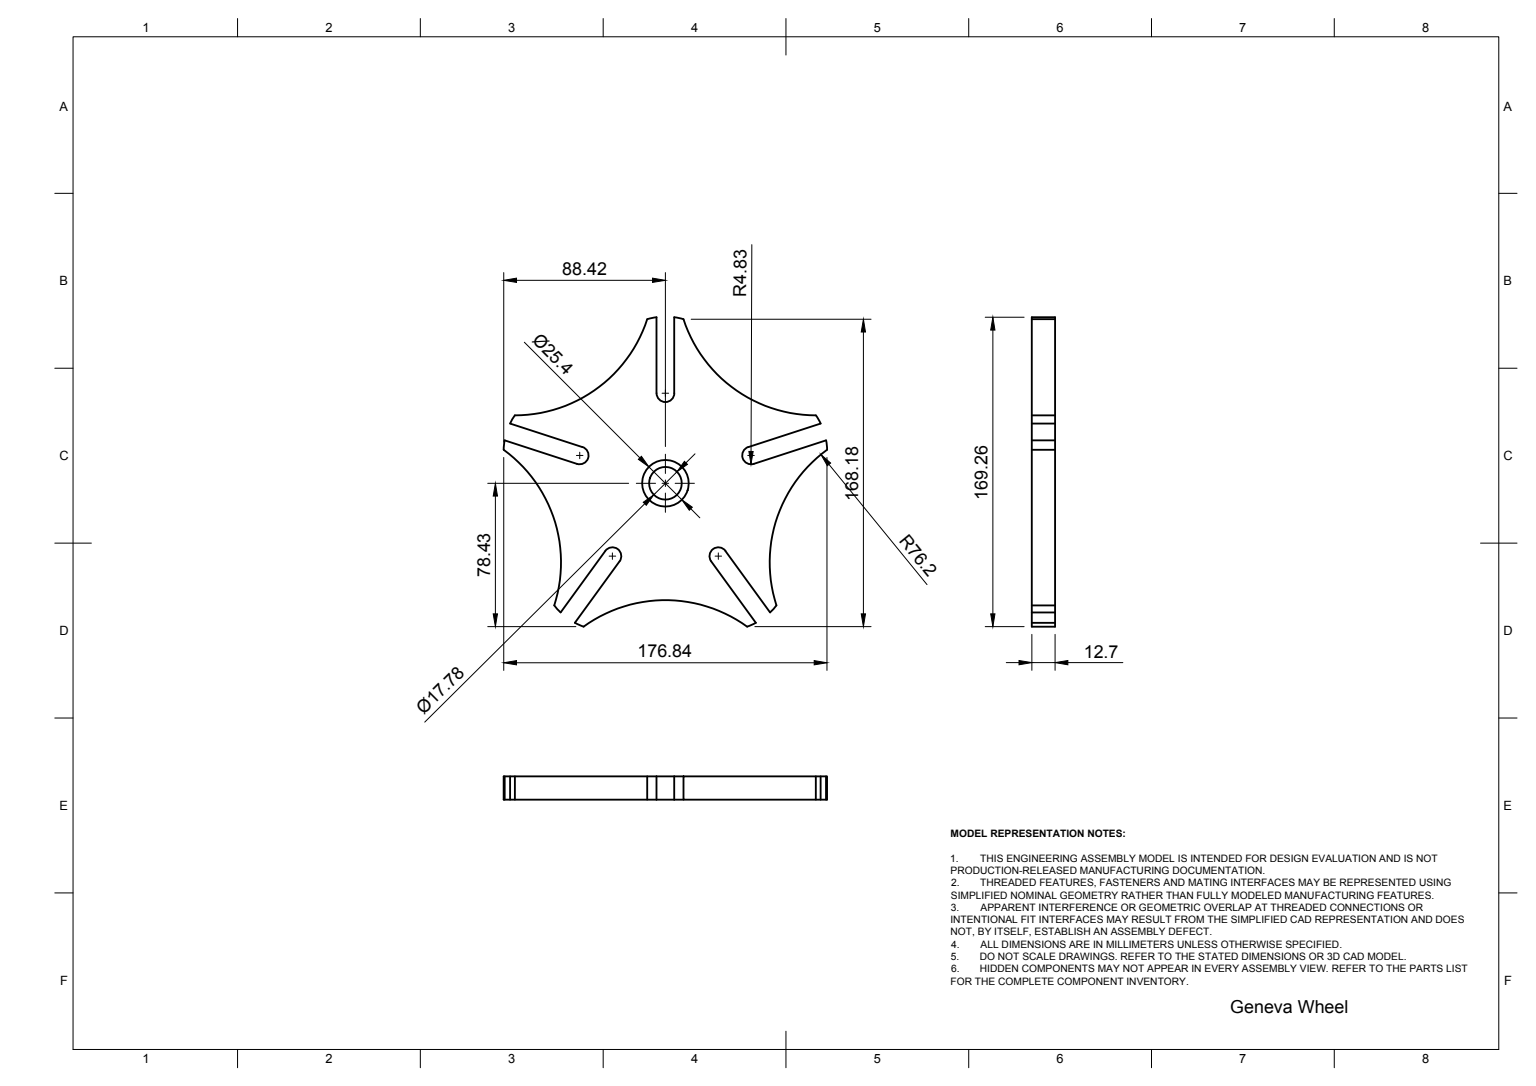
ISO-10303-21;
HEADER;
/* Generated by software containing ST-Developer
 * from STEP Tools, Inc. (www.steptools.com) 
 */

FILE_DESCRIPTION(
/* description */ ('STEP AP214'),
/* implementation_level */ '2;1');

FILE_NAME(
/* name */ 'Geneva Wheel.step',
/* time_stamp */ '2026-10-06T11:20:11-07:00',
/* author */ (''),
/* organization */ (''),
/* preprocessor_version */ 'ST-DEVELOPER v20.2',
/* originating_system */ 'Autodesk Translation Framework v15.15.0.0',
/* authorisation */ '');

FILE_SCHEMA (('AUTOMOTIVE_DESIGN { 1 0 10303 214 3 1 1 }'));
ENDSEC;

DATA;
#10=MECHANICAL_DESIGN_GEOMETRIC_PRESENTATION_REPRESENTATION('',(#51),#2840);
#39=SHAPE_REPRESENTATION_RELATIONSHIP('SRR','None',#2870,#45);
#45=ADVANCED_BREP_SHAPE_REPRESENTATION('',(#57),#2838);
#51=STYLED_ITEM('',(#2905),#57);
#57=MANIFOLD_SOLID_BREP('Body1',#1551);
#95=FACE_BOUND('',#299,.T.);
#96=FACE_BOUND('',#301,.T.);
#97=FACE_BOUND('',#330,.T.);
#111=PLANE('',#1765);
#112=PLANE('',#1783);
#113=PLANE('',#1802);
#114=PLANE('',#1806);
#115=PLANE('',#1808);
#116=PLANE('',#1812);
#117=PLANE('',#1813);
#118=PLANE('',#1816);
#119=PLANE('',#1817);
#120=PLANE('',#1821);
#121=PLANE('',#1823);
#122=PLANE('',#1827);
#123=PLANE('',#1828);
#178=FACE_OUTER_BOUND('',#293,.T.);
#179=FACE_OUTER_BOUND('',#294,.T.);
#180=FACE_OUTER_BOUND('',#295,.T.);
#181=FACE_OUTER_BOUND('',#296,.T.);
#182=FACE_OUTER_BOUND('',#297,.T.);
#183=FACE_OUTER_BOUND('',#298,.T.);
#184=FACE_OUTER_BOUND('',#300,.T.);
#185=FACE_OUTER_BOUND('',#302,.T.);
#186=FACE_OUTER_BOUND('',#303,.T.);
#187=FACE_OUTER_BOUND('',#304,.T.);
#188=FACE_OUTER_BOUND('',#305,.T.);
#189=FACE_OUTER_BOUND('',#306,.T.);
#190=FACE_OUTER_BOUND('',#307,.T.);
#191=FACE_OUTER_BOUND('',#308,.T.);
#192=FACE_OUTER_BOUND('',#309,.T.);
#193=FACE_OUTER_BOUND('',#310,.T.);
#194=FACE_OUTER_BOUND('',#311,.T.);
#195=FACE_OUTER_BOUND('',#312,.T.);
#196=FACE_OUTER_BOUND('',#313,.T.);
#197=FACE_OUTER_BOUND('',#314,.T.);
#198=FACE_OUTER_BOUND('',#315,.T.);
#199=FACE_OUTER_BOUND('',#316,.T.);
#200=FACE_OUTER_BOUND('',#317,.T.);
#201=FACE_OUTER_BOUND('',#318,.T.);
#202=FACE_OUTER_BOUND('',#319,.T.);
#203=FACE_OUTER_BOUND('',#320,.T.);
#204=FACE_OUTER_BOUND('',#321,.T.);
#205=FACE_OUTER_BOUND('',#322,.T.);
#206=FACE_OUTER_BOUND('',#323,.T.);
#207=FACE_OUTER_BOUND('',#324,.T.);
#208=FACE_OUTER_BOUND('',#325,.T.);
#209=FACE_OUTER_BOUND('',#326,.T.);
#210=FACE_OUTER_BOUND('',#327,.T.);
#211=FACE_OUTER_BOUND('',#328,.T.);
#212=FACE_OUTER_BOUND('',#329,.T.);
#293=EDGE_LOOP('',(#1208,#1209,#1210,#1211));
#294=EDGE_LOOP('',(#1212,#1213,#1214,#1215));
#295=EDGE_LOOP('',(#1216,#1217,#1218,#1219));
#296=EDGE_LOOP('',(#1220,#1221,#1222,#1223));
#297=EDGE_LOOP('',(#1224,#1225,#1226,#1227));
#298=EDGE_LOOP('',(#1228,#1229,#1230,#1231,#1232,#1233,#1234,#1235,#1236,
#1237,#1238,#1239,#1240,#1241,#1242,#1243,#1244,#1245,#1246,#1247,#1248,
#1249,#1250,#1251,#1252,#1253,#1254,#1255,#1256,#1257));
#299=EDGE_LOOP('',(#1258));
#300=EDGE_LOOP('',(#1259,#1260,#1261,#1262,#1263,#1264,#1265,#1266,#1267,
#1268,#1269,#1270,#1271,#1272,#1273,#1274,#1275,#1276,#1277,#1278,#1279,
#1280,#1281,#1282,#1283,#1284,#1285,#1286,#1287,#1288));
#301=EDGE_LOOP('',(#1289));
#302=EDGE_LOOP('',(#1290,#1291,#1292,#1293));
#303=EDGE_LOOP('',(#1294,#1295,#1296,#1297));
#304=EDGE_LOOP('',(#1298,#1299,#1300,#1301));
#305=EDGE_LOOP('',(#1302,#1303,#1304,#1305));
#306=EDGE_LOOP('',(#1306,#1307,#1308,#1309));
#307=EDGE_LOOP('',(#1310,#1311,#1312,#1313));
#308=EDGE_LOOP('',(#1314,#1315,#1316,#1317));
#309=EDGE_LOOP('',(#1318,#1319,#1320,#1321));
#310=EDGE_LOOP('',(#1322,#1323,#1324,#1325));
#311=EDGE_LOOP('',(#1326,#1327,#1328,#1329));
#312=EDGE_LOOP('',(#1330,#1331,#1332,#1333));
#313=EDGE_LOOP('',(#1334,#1335,#1336,#1337));
#314=EDGE_LOOP('',(#1338,#1339,#1340,#1341));
#315=EDGE_LOOP('',(#1342,#1343,#1344,#1345));
#316=EDGE_LOOP('',(#1346,#1347,#1348,#1349));
#317=EDGE_LOOP('',(#1350,#1351,#1352,#1353));
#318=EDGE_LOOP('',(#1354,#1355,#1356,#1357));
#319=EDGE_LOOP('',(#1358,#1359,#1360,#1361));
#320=EDGE_LOOP('',(#1362,#1363,#1364,#1365));
#321=EDGE_LOOP('',(#1366,#1367,#1368,#1369));
#322=EDGE_LOOP('',(#1370,#1371,#1372,#1373));
#323=EDGE_LOOP('',(#1374,#1375,#1376,#1377));
#324=EDGE_LOOP('',(#1378,#1379,#1380,#1381));
#325=EDGE_LOOP('',(#1382,#1383,#1384,#1385));
#326=EDGE_LOOP('',(#1386,#1387,#1388,#1389));
#327=EDGE_LOOP('',(#1390,#1391,#1392,#1393));
#328=EDGE_LOOP('',(#1394,#1395,#1396,#1397));
#329=EDGE_LOOP('',(#1398));
#330=EDGE_LOOP('',(#1399));
#374=LINE('',#2619,#467);
#375=LINE('',#2626,#468);
#376=LINE('',#2629,#469);
#377=LINE('',#2635,#470);
#378=LINE('',#2638,#471);
#379=LINE('',#2644,#472);
#380=LINE('',#2647,#473);
#381=LINE('',#2652,#474);
#382=LINE('',#2659,#475);
#383=LINE('',#2667,#476);
#384=LINE('',#2671,#477);
#385=LINE('',#2678,#478);
#386=LINE('',#2680,#479);
#387=LINE('',#2684,#480);
#388=LINE('',#2686,#481);
#389=LINE('',#2694,#482);
#390=LINE('',#2698,#483);
#391=LINE('',#2705,#484);
#392=LINE('',#2711,#485);
#393=LINE('',#2719,#486);
#394=LINE('',#2723,#487);
#395=LINE('',#2730,#488);
#396=LINE('',#2732,#489);
#397=LINE('',#2736,#490);
#398=LINE('',#2738,#491);
#399=LINE('',#2746,#492);
#400=LINE('',#2750,#493);
#401=LINE('',#2757,#494);
#402=LINE('',#2759,#495);
#403=LINE('',#2760,#496);
#404=LINE('',#2762,#497);
#405=LINE('',#2764,#498);
#406=LINE('',#2766,#499);
#407=LINE('',#2768,#500);
#408=LINE('',#2770,#501);
#409=LINE('',#2772,#502);
#410=LINE('',#2774,#503);
#411=LINE('',#2776,#504);
#412=LINE('',#2778,#505);
#413=LINE('',#2780,#506);
#414=LINE('',#2783,#507);
#415=LINE('',#2786,#508);
#416=LINE('',#2789,#509);
#417=LINE('',#2791,#510);
#418=LINE('',#2793,#511);
#419=LINE('',#2795,#512);
#420=LINE('',#2797,#513);
#421=LINE('',#2799,#514);
#422=LINE('',#2801,#515);
#423=LINE('',#2803,#516);
#424=LINE('',#2805,#517);
#425=LINE('',#2807,#518);
#467=VECTOR('',#2145,12.7);
#468=VECTOR('',#2152,1000.);
#469=VECTOR('',#2155,1000.);
#470=VECTOR('',#2160,1000.);
#471=VECTOR('',#2163,1000.);
#472=VECTOR('',#2168,1000.);
#473=VECTOR('',#2171,1000.);
#474=VECTOR('',#2176,8.88999999999999);
#475=VECTOR('',#2183,1000.);
#476=VECTOR('',#2190,1000.);
#477=VECTOR('',#2193,1000.);
#478=VECTOR('',#2200,1000.);
#479=VECTOR('',#2201,1000.);
#480=VECTOR('',#2206,1000.);
#481=VECTOR('',#2207,1000.);
#482=VECTOR('',#2214,1000.);
#483=VECTOR('',#2217,1000.);
#484=VECTOR('',#2224,1000.);
#485=VECTOR('',#2229,1000.);
#486=VECTOR('',#2236,1000.);
#487=VECTOR('',#2239,1000.);
#488=VECTOR('',#2246,1000.);
#489=VECTOR('',#2247,1000.);
#490=VECTOR('',#2252,1000.);
#491=VECTOR('',#2253,1000.);
#492=VECTOR('',#2260,1000.);
#493=VECTOR('',#2263,1000.);
#494=VECTOR('',#2270,1000.);
#495=VECTOR('',#2273,1000.);
#496=VECTOR('',#2274,1000.);
#497=VECTOR('',#2277,1000.);
#498=VECTOR('',#2280,1000.);
#499=VECTOR('',#2283,1000.);
#500=VECTOR('',#2286,1000.);
#501=VECTOR('',#2289,1000.);
#502=VECTOR('',#2292,1000.);
#503=VECTOR('',#2295,1000.);
#504=VECTOR('',#2298,1000.);
#505=VECTOR('',#2301,1000.);
#506=VECTOR('',#2304,1000.);
#507=VECTOR('',#2309,1000.);
#508=VECTOR('',#2314,1000.);
#509=VECTOR('',#2319,1000.);
#510=VECTOR('',#2322,1000.);
#511=VECTOR('',#2325,1000.);
#512=VECTOR('',#2328,1000.);
#513=VECTOR('',#2331,1000.);
#514=VECTOR('',#2334,1000.);
#515=VECTOR('',#2337,1000.);
#516=VECTOR('',#2340,1000.);
#517=VECTOR('',#2343,1000.);
#518=VECTOR('',#2346,1000.);
#592=CIRCLE('',#1751,12.7);
#593=CIRCLE('',#1752,12.7);
#594=CIRCLE('',#1754,4.826);
#595=CIRCLE('',#1755,4.826);
#596=CIRCLE('',#1757,76.1999999999999);
#597=CIRCLE('',#1758,76.1999999999999);
#598=CIRCLE('',#1760,4.826);
#599=CIRCLE('',#1761,4.826);
#600=CIRCLE('',#1763,8.88999999999999);
#601=CIRCLE('',#1764,8.88999999999999);
#602=CIRCLE('',#1766,4.826);
#603=CIRCLE('',#1767,27.0465001077289);
#604=CIRCLE('',#1768,76.2);
#605=CIRCLE('',#1769,27.0465001077289);
#606=CIRCLE('',#1770,4.826);
#607=CIRCLE('',#1771,27.0465001077289);
#608=CIRCLE('',#1772,76.1999999999999);
#609=CIRCLE('',#1773,27.0465001077289);
#610=CIRCLE('',#1774,27.0465001077289);
#611=CIRCLE('',#1775,27.0465001077289);
#612=CIRCLE('',#1776,27.0465001077289);
#613=CIRCLE('',#1777,76.1999999999999);
#614=CIRCLE('',#1778,27.0465001077289);
#615=CIRCLE('',#1779,4.826);
#616=CIRCLE('',#1780,27.0465001077289);
#617=CIRCLE('',#1781,76.1999999999999);
#618=CIRCLE('',#1782,27.0465001077289);
#619=CIRCLE('',#1784,4.826);
#620=CIRCLE('',#1785,27.0465001077289);
#621=CIRCLE('',#1786,76.1999999999999);
#622=CIRCLE('',#1787,27.0465001077289);
#623=CIRCLE('',#1788,4.826);
#624=CIRCLE('',#1789,27.0465001077289);
#625=CIRCLE('',#1790,76.1999999999999);
#626=CIRCLE('',#1791,27.0465001077289);
#627=CIRCLE('',#1792,27.0465001077289);
#628=CIRCLE('',#1793,27.0465001077289);
#629=CIRCLE('',#1794,27.0465001077289);
#630=CIRCLE('',#1795,76.1999999999999);
#631=CIRCLE('',#1796,27.0465001077289);
#632=CIRCLE('',#1797,4.826);
#633=CIRCLE('',#1798,27.0465001077289);
#634=CIRCLE('',#1799,76.2);
#635=CIRCLE('',#1800,27.0465001077289);
#707=VERTEX_POINT('',#2616);
#708=VERTEX_POINT('',#2618);
#709=VERTEX_POINT('',#2622);
#710=VERTEX_POINT('',#2623);
#711=VERTEX_POINT('',#2625);
#712=VERTEX_POINT('',#2627);
#713=VERTEX_POINT('',#2631);
#714=VERTEX_POINT('',#2632);
#715=VERTEX_POINT('',#2634);
#716=VERTEX_POINT('',#2636);
#717=VERTEX_POINT('',#2640);
#718=VERTEX_POINT('',#2641);
#719=VERTEX_POINT('',#2643);
#720=VERTEX_POINT('',#2645);
#721=VERTEX_POINT('',#2649);
#722=VERTEX_POINT('',#2651);
#723=VERTEX_POINT('',#2655);
#724=VERTEX_POINT('',#2656);
#725=VERTEX_POINT('',#2658);
#726=VERTEX_POINT('',#2660);
#727=VERTEX_POINT('',#2662);
#728=VERTEX_POINT('',#2664);
#729=VERTEX_POINT('',#2666);
#730=VERTEX_POINT('',#2668);
#731=VERTEX_POINT('',#2670);
#732=VERTEX_POINT('',#2672);
#733=VERTEX_POINT('',#2674);
#734=VERTEX_POINT('',#2676);
#735=VERTEX_POINT('',#2679);
#736=VERTEX_POINT('',#2682);
#737=VERTEX_POINT('',#2685);
#738=VERTEX_POINT('',#2687);
#739=VERTEX_POINT('',#2689);
#740=VERTEX_POINT('',#2691);
#741=VERTEX_POINT('',#2693);
#742=VERTEX_POINT('',#2695);
#743=VERTEX_POINT('',#2697);
#744=VERTEX_POINT('',#2699);
#745=VERTEX_POINT('',#2701);
#746=VERTEX_POINT('',#2703);
#747=VERTEX_POINT('',#2707);
#748=VERTEX_POINT('',#2708);
#749=VERTEX_POINT('',#2710);
#750=VERTEX_POINT('',#2712);
#751=VERTEX_POINT('',#2714);
#752=VERTEX_POINT('',#2716);
#753=VERTEX_POINT('',#2718);
#754=VERTEX_POINT('',#2720);
#755=VERTEX_POINT('',#2722);
#756=VERTEX_POINT('',#2724);
#757=VERTEX_POINT('',#2726);
#758=VERTEX_POINT('',#2728);
#759=VERTEX_POINT('',#2731);
#760=VERTEX_POINT('',#2734);
#761=VERTEX_POINT('',#2737);
#762=VERTEX_POINT('',#2739);
#763=VERTEX_POINT('',#2741);
#764=VERTEX_POINT('',#2743);
#765=VERTEX_POINT('',#2745);
#766=VERTEX_POINT('',#2747);
#767=VERTEX_POINT('',#2749);
#768=VERTEX_POINT('',#2751);
#769=VERTEX_POINT('',#2753);
#770=VERTEX_POINT('',#2755);
#885=EDGE_CURVE('',#707,#707,#592,.T.);
#886=EDGE_CURVE('',#707,#708,#374,.T.);
#887=EDGE_CURVE('',#708,#708,#593,.T.);
#888=EDGE_CURVE('',#709,#710,#594,.T.);
#889=EDGE_CURVE('',#709,#711,#375,.T.);
#890=EDGE_CURVE('',#711,#712,#595,.T.);
#891=EDGE_CURVE('',#710,#712,#376,.T.);
#892=EDGE_CURVE('',#713,#714,#596,.T.);
#893=EDGE_CURVE('',#713,#715,#377,.T.);
#894=EDGE_CURVE('',#715,#716,#597,.T.);
#895=EDGE_CURVE('',#714,#716,#378,.T.);
#896=EDGE_CURVE('',#717,#718,#598,.T.);
#897=EDGE_CURVE('',#717,#719,#379,.T.);
#898=EDGE_CURVE('',#719,#720,#599,.T.);
#899=EDGE_CURVE('',#718,#720,#380,.T.);
#900=EDGE_CURVE('',#721,#721,#600,.T.);
#901=EDGE_CURVE('',#721,#722,#381,.T.);
#902=EDGE_CURVE('',#722,#722,#601,.T.);
#903=EDGE_CURVE('',#723,#724,#602,.T.);
#904=EDGE_CURVE('',#724,#725,#382,.T.);
#905=EDGE_CURVE('',#725,#726,#603,.T.);
#906=EDGE_CURVE('',#726,#727,#604,.T.);
#907=EDGE_CURVE('',#727,#728,#605,.T.);
#908=EDGE_CURVE('',#728,#729,#383,.T.);
#909=EDGE_CURVE('',#729,#730,#606,.T.);
#910=EDGE_CURVE('',#730,#731,#384,.T.);
#911=EDGE_CURVE('',#731,#732,#607,.T.);
#912=EDGE_CURVE('',#732,#733,#608,.T.);
#913=EDGE_CURVE('',#733,#734,#609,.T.);
#914=EDGE_CURVE('',#734,#717,#385,.T.);
#915=EDGE_CURVE('',#718,#735,#386,.T.);
#916=EDGE_CURVE('',#735,#713,#610,.T.);
#917=EDGE_CURVE('',#714,#736,#611,.T.);
#918=EDGE_CURVE('',#736,#709,#387,.T.);
#919=EDGE_CURVE('',#710,#737,#388,.T.);
#920=EDGE_CURVE('',#737,#738,#612,.T.);
#921=EDGE_CURVE('',#738,#739,#613,.T.);
#922=EDGE_CURVE('',#739,#740,#614,.T.);
#923=EDGE_CURVE('',#740,#741,#389,.T.);
#924=EDGE_CURVE('',#741,#742,#615,.T.);
#925=EDGE_CURVE('',#742,#743,#390,.T.);
#926=EDGE_CURVE('',#743,#744,#616,.T.);
#927=EDGE_CURVE('',#744,#745,#617,.T.);
#928=EDGE_CURVE('',#745,#746,#618,.T.);
#929=EDGE_CURVE('',#746,#723,#391,.T.);
#930=EDGE_CURVE('',#747,#748,#619,.T.);
#931=EDGE_CURVE('',#749,#747,#392,.T.);
#932=EDGE_CURVE('',#750,#749,#620,.T.);
#933=EDGE_CURVE('',#751,#750,#621,.T.);
#934=EDGE_CURVE('',#752,#751,#622,.T.);
#935=EDGE_CURVE('',#753,#752,#393,.T.);
#936=EDGE_CURVE('',#754,#753,#623,.T.);
#937=EDGE_CURVE('',#755,#754,#394,.T.);
#938=EDGE_CURVE('',#756,#755,#624,.T.);
#939=EDGE_CURVE('',#757,#756,#625,.T.);
#940=EDGE_CURVE('',#758,#757,#626,.T.);
#941=EDGE_CURVE('',#712,#758,#395,.T.);
#942=EDGE_CURVE('',#759,#711,#396,.T.);
#943=EDGE_CURVE('',#716,#759,#627,.T.);
#944=EDGE_CURVE('',#760,#715,#628,.T.);
#945=EDGE_CURVE('',#720,#760,#397,.T.);
#946=EDGE_CURVE('',#761,#719,#398,.T.);
#947=EDGE_CURVE('',#762,#761,#629,.T.);
#948=EDGE_CURVE('',#763,#762,#630,.T.);
#949=EDGE_CURVE('',#764,#763,#631,.T.);
#950=EDGE_CURVE('',#765,#764,#399,.T.);
#951=EDGE_CURVE('',#766,#765,#632,.T.);
#952=EDGE_CURVE('',#767,#766,#400,.T.);
#953=EDGE_CURVE('',#768,#767,#633,.T.);
#954=EDGE_CURVE('',#769,#768,#634,.T.);
#955=EDGE_CURVE('',#770,#769,#635,.T.);
#956=EDGE_CURVE('',#748,#770,#401,.T.);
#957=EDGE_CURVE('',#724,#748,#402,.T.);
#958=EDGE_CURVE('',#723,#747,#403,.T.);
#959=EDGE_CURVE('',#725,#770,#404,.T.);
#960=EDGE_CURVE('',#726,#769,#405,.T.);
#961=EDGE_CURVE('',#727,#768,#406,.T.);
#962=EDGE_CURVE('',#728,#767,#407,.T.);
#963=EDGE_CURVE('',#729,#766,#408,.T.);
#964=EDGE_CURVE('',#730,#765,#409,.T.);
#965=EDGE_CURVE('',#731,#764,#410,.T.);
#966=EDGE_CURVE('',#732,#763,#411,.T.);
#967=EDGE_CURVE('',#733,#762,#412,.T.);
#968=EDGE_CURVE('',#734,#761,#413,.T.);
#969=EDGE_CURVE('',#735,#760,#414,.T.);
#970=EDGE_CURVE('',#736,#759,#415,.T.);
#971=EDGE_CURVE('',#737,#758,#416,.T.);
#972=EDGE_CURVE('',#738,#757,#417,.T.);
#973=EDGE_CURVE('',#739,#756,#418,.T.);
#974=EDGE_CURVE('',#740,#755,#419,.T.);
#975=EDGE_CURVE('',#741,#754,#420,.T.);
#976=EDGE_CURVE('',#742,#753,#421,.T.);
#977=EDGE_CURVE('',#743,#752,#422,.T.);
#978=EDGE_CURVE('',#744,#751,#423,.T.);
#979=EDGE_CURVE('',#745,#750,#424,.T.);
#980=EDGE_CURVE('',#746,#749,#425,.T.);
#1208=ORIENTED_EDGE('',*,*,#885,.F.);
#1209=ORIENTED_EDGE('',*,*,#886,.T.);
#1210=ORIENTED_EDGE('',*,*,#887,.T.);
#1211=ORIENTED_EDGE('',*,*,#886,.F.);
#1212=ORIENTED_EDGE('',*,*,#888,.F.);
#1213=ORIENTED_EDGE('',*,*,#889,.T.);
#1214=ORIENTED_EDGE('',*,*,#890,.T.);
#1215=ORIENTED_EDGE('',*,*,#891,.F.);
#1216=ORIENTED_EDGE('',*,*,#892,.F.);
#1217=ORIENTED_EDGE('',*,*,#893,.T.);
#1218=ORIENTED_EDGE('',*,*,#894,.T.);
#1219=ORIENTED_EDGE('',*,*,#895,.F.);
#1220=ORIENTED_EDGE('',*,*,#896,.F.);
#1221=ORIENTED_EDGE('',*,*,#897,.T.);
#1222=ORIENTED_EDGE('',*,*,#898,.T.);
#1223=ORIENTED_EDGE('',*,*,#899,.F.);
#1224=ORIENTED_EDGE('',*,*,#900,.F.);
#1225=ORIENTED_EDGE('',*,*,#901,.T.);
#1226=ORIENTED_EDGE('',*,*,#902,.T.);
#1227=ORIENTED_EDGE('',*,*,#901,.F.);
#1228=ORIENTED_EDGE('',*,*,#903,.T.);
#1229=ORIENTED_EDGE('',*,*,#904,.T.);
#1230=ORIENTED_EDGE('',*,*,#905,.T.);
#1231=ORIENTED_EDGE('',*,*,#906,.T.);
#1232=ORIENTED_EDGE('',*,*,#907,.T.);
#1233=ORIENTED_EDGE('',*,*,#908,.T.);
#1234=ORIENTED_EDGE('',*,*,#909,.T.);
#1235=ORIENTED_EDGE('',*,*,#910,.T.);
#1236=ORIENTED_EDGE('',*,*,#911,.T.);
#1237=ORIENTED_EDGE('',*,*,#912,.T.);
#1238=ORIENTED_EDGE('',*,*,#913,.T.);
#1239=ORIENTED_EDGE('',*,*,#914,.T.);
#1240=ORIENTED_EDGE('',*,*,#896,.T.);
#1241=ORIENTED_EDGE('',*,*,#915,.T.);
#1242=ORIENTED_EDGE('',*,*,#916,.T.);
#1243=ORIENTED_EDGE('',*,*,#892,.T.);
#1244=ORIENTED_EDGE('',*,*,#917,.T.);
#1245=ORIENTED_EDGE('',*,*,#918,.T.);
#1246=ORIENTED_EDGE('',*,*,#888,.T.);
#1247=ORIENTED_EDGE('',*,*,#919,.T.);
#1248=ORIENTED_EDGE('',*,*,#920,.T.);
#1249=ORIENTED_EDGE('',*,*,#921,.T.);
#1250=ORIENTED_EDGE('',*,*,#922,.T.);
#1251=ORIENTED_EDGE('',*,*,#923,.T.);
#1252=ORIENTED_EDGE('',*,*,#924,.T.);
#1253=ORIENTED_EDGE('',*,*,#925,.T.);
#1254=ORIENTED_EDGE('',*,*,#926,.T.);
#1255=ORIENTED_EDGE('',*,*,#927,.T.);
#1256=ORIENTED_EDGE('',*,*,#928,.T.);
#1257=ORIENTED_EDGE('',*,*,#929,.T.);
#1258=ORIENTED_EDGE('',*,*,#887,.F.);
#1259=ORIENTED_EDGE('',*,*,#930,.F.);
#1260=ORIENTED_EDGE('',*,*,#931,.F.);
#1261=ORIENTED_EDGE('',*,*,#932,.F.);
#1262=ORIENTED_EDGE('',*,*,#933,.F.);
#1263=ORIENTED_EDGE('',*,*,#934,.F.);
#1264=ORIENTED_EDGE('',*,*,#935,.F.);
#1265=ORIENTED_EDGE('',*,*,#936,.F.);
#1266=ORIENTED_EDGE('',*,*,#937,.F.);
#1267=ORIENTED_EDGE('',*,*,#938,.F.);
#1268=ORIENTED_EDGE('',*,*,#939,.F.);
#1269=ORIENTED_EDGE('',*,*,#940,.F.);
#1270=ORIENTED_EDGE('',*,*,#941,.F.);
#1271=ORIENTED_EDGE('',*,*,#890,.F.);
#1272=ORIENTED_EDGE('',*,*,#942,.F.);
#1273=ORIENTED_EDGE('',*,*,#943,.F.);
#1274=ORIENTED_EDGE('',*,*,#894,.F.);
#1275=ORIENTED_EDGE('',*,*,#944,.F.);
#1276=ORIENTED_EDGE('',*,*,#945,.F.);
#1277=ORIENTED_EDGE('',*,*,#898,.F.);
#1278=ORIENTED_EDGE('',*,*,#946,.F.);
#1279=ORIENTED_EDGE('',*,*,#947,.F.);
#1280=ORIENTED_EDGE('',*,*,#948,.F.);
#1281=ORIENTED_EDGE('',*,*,#949,.F.);
#1282=ORIENTED_EDGE('',*,*,#950,.F.);
#1283=ORIENTED_EDGE('',*,*,#951,.F.);
#1284=ORIENTED_EDGE('',*,*,#952,.F.);
#1285=ORIENTED_EDGE('',*,*,#953,.F.);
#1286=ORIENTED_EDGE('',*,*,#954,.F.);
#1287=ORIENTED_EDGE('',*,*,#955,.F.);
#1288=ORIENTED_EDGE('',*,*,#956,.F.);
#1289=ORIENTED_EDGE('',*,*,#902,.F.);
#1290=ORIENTED_EDGE('',*,*,#930,.T.);
#1291=ORIENTED_EDGE('',*,*,#957,.F.);
#1292=ORIENTED_EDGE('',*,*,#903,.F.);
#1293=ORIENTED_EDGE('',*,*,#958,.T.);
#1294=ORIENTED_EDGE('',*,*,#956,.T.);
#1295=ORIENTED_EDGE('',*,*,#959,.F.);
#1296=ORIENTED_EDGE('',*,*,#904,.F.);
#1297=ORIENTED_EDGE('',*,*,#957,.T.);
#1298=ORIENTED_EDGE('',*,*,#955,.T.);
#1299=ORIENTED_EDGE('',*,*,#960,.F.);
#1300=ORIENTED_EDGE('',*,*,#905,.F.);
#1301=ORIENTED_EDGE('',*,*,#959,.T.);
#1302=ORIENTED_EDGE('',*,*,#954,.T.);
#1303=ORIENTED_EDGE('',*,*,#961,.F.);
#1304=ORIENTED_EDGE('',*,*,#906,.F.);
#1305=ORIENTED_EDGE('',*,*,#960,.T.);
#1306=ORIENTED_EDGE('',*,*,#953,.T.);
#1307=ORIENTED_EDGE('',*,*,#962,.F.);
#1308=ORIENTED_EDGE('',*,*,#907,.F.);
#1309=ORIENTED_EDGE('',*,*,#961,.T.);
#1310=ORIENTED_EDGE('',*,*,#952,.T.);
#1311=ORIENTED_EDGE('',*,*,#963,.F.);
#1312=ORIENTED_EDGE('',*,*,#908,.F.);
#1313=ORIENTED_EDGE('',*,*,#962,.T.);
#1314=ORIENTED_EDGE('',*,*,#951,.T.);
#1315=ORIENTED_EDGE('',*,*,#964,.F.);
#1316=ORIENTED_EDGE('',*,*,#909,.F.);
#1317=ORIENTED_EDGE('',*,*,#963,.T.);
#1318=ORIENTED_EDGE('',*,*,#950,.T.);
#1319=ORIENTED_EDGE('',*,*,#965,.F.);
#1320=ORIENTED_EDGE('',*,*,#910,.F.);
#1321=ORIENTED_EDGE('',*,*,#964,.T.);
#1322=ORIENTED_EDGE('',*,*,#949,.T.);
#1323=ORIENTED_EDGE('',*,*,#966,.F.);
#1324=ORIENTED_EDGE('',*,*,#911,.F.);
#1325=ORIENTED_EDGE('',*,*,#965,.T.);
#1326=ORIENTED_EDGE('',*,*,#948,.T.);
#1327=ORIENTED_EDGE('',*,*,#967,.F.);
#1328=ORIENTED_EDGE('',*,*,#912,.F.);
#1329=ORIENTED_EDGE('',*,*,#966,.T.);
#1330=ORIENTED_EDGE('',*,*,#947,.T.);
#1331=ORIENTED_EDGE('',*,*,#968,.F.);
#1332=ORIENTED_EDGE('',*,*,#913,.F.);
#1333=ORIENTED_EDGE('',*,*,#967,.T.);
#1334=ORIENTED_EDGE('',*,*,#946,.T.);
#1335=ORIENTED_EDGE('',*,*,#897,.F.);
#1336=ORIENTED_EDGE('',*,*,#914,.F.);
#1337=ORIENTED_EDGE('',*,*,#968,.T.);
#1338=ORIENTED_EDGE('',*,*,#945,.T.);
#1339=ORIENTED_EDGE('',*,*,#969,.F.);
#1340=ORIENTED_EDGE('',*,*,#915,.F.);
#1341=ORIENTED_EDGE('',*,*,#899,.T.);
#1342=ORIENTED_EDGE('',*,*,#944,.T.);
#1343=ORIENTED_EDGE('',*,*,#893,.F.);
#1344=ORIENTED_EDGE('',*,*,#916,.F.);
#1345=ORIENTED_EDGE('',*,*,#969,.T.);
#1346=ORIENTED_EDGE('',*,*,#943,.T.);
#1347=ORIENTED_EDGE('',*,*,#970,.F.);
#1348=ORIENTED_EDGE('',*,*,#917,.F.);
#1349=ORIENTED_EDGE('',*,*,#895,.T.);
#1350=ORIENTED_EDGE('',*,*,#942,.T.);
#1351=ORIENTED_EDGE('',*,*,#889,.F.);
#1352=ORIENTED_EDGE('',*,*,#918,.F.);
#1353=ORIENTED_EDGE('',*,*,#970,.T.);
#1354=ORIENTED_EDGE('',*,*,#941,.T.);
#1355=ORIENTED_EDGE('',*,*,#971,.F.);
#1356=ORIENTED_EDGE('',*,*,#919,.F.);
#1357=ORIENTED_EDGE('',*,*,#891,.T.);
#1358=ORIENTED_EDGE('',*,*,#940,.T.);
#1359=ORIENTED_EDGE('',*,*,#972,.F.);
#1360=ORIENTED_EDGE('',*,*,#920,.F.);
#1361=ORIENTED_EDGE('',*,*,#971,.T.);
#1362=ORIENTED_EDGE('',*,*,#939,.T.);
#1363=ORIENTED_EDGE('',*,*,#973,.F.);
#1364=ORIENTED_EDGE('',*,*,#921,.F.);
#1365=ORIENTED_EDGE('',*,*,#972,.T.);
#1366=ORIENTED_EDGE('',*,*,#938,.T.);
#1367=ORIENTED_EDGE('',*,*,#974,.F.);
#1368=ORIENTED_EDGE('',*,*,#922,.F.);
#1369=ORIENTED_EDGE('',*,*,#973,.T.);
#1370=ORIENTED_EDGE('',*,*,#937,.T.);
#1371=ORIENTED_EDGE('',*,*,#975,.F.);
#1372=ORIENTED_EDGE('',*,*,#923,.F.);
#1373=ORIENTED_EDGE('',*,*,#974,.T.);
#1374=ORIENTED_EDGE('',*,*,#936,.T.);
#1375=ORIENTED_EDGE('',*,*,#976,.F.);
#1376=ORIENTED_EDGE('',*,*,#924,.F.);
#1377=ORIENTED_EDGE('',*,*,#975,.T.);
#1378=ORIENTED_EDGE('',*,*,#935,.T.);
#1379=ORIENTED_EDGE('',*,*,#977,.F.);
#1380=ORIENTED_EDGE('',*,*,#925,.F.);
#1381=ORIENTED_EDGE('',*,*,#976,.T.);
#1382=ORIENTED_EDGE('',*,*,#934,.T.);
#1383=ORIENTED_EDGE('',*,*,#978,.F.);
#1384=ORIENTED_EDGE('',*,*,#926,.F.);
#1385=ORIENTED_EDGE('',*,*,#977,.T.);
#1386=ORIENTED_EDGE('',*,*,#933,.T.);
#1387=ORIENTED_EDGE('',*,*,#979,.F.);
#1388=ORIENTED_EDGE('',*,*,#927,.F.);
#1389=ORIENTED_EDGE('',*,*,#978,.T.);
#1390=ORIENTED_EDGE('',*,*,#932,.T.);
#1391=ORIENTED_EDGE('',*,*,#980,.F.);
#1392=ORIENTED_EDGE('',*,*,#928,.F.);
#1393=ORIENTED_EDGE('',*,*,#979,.T.);
#1394=ORIENTED_EDGE('',*,*,#931,.T.);
#1395=ORIENTED_EDGE('',*,*,#958,.F.);
#1396=ORIENTED_EDGE('',*,*,#929,.F.);
#1397=ORIENTED_EDGE('',*,*,#980,.T.);
#1398=ORIENTED_EDGE('',*,*,#885,.T.);
#1399=ORIENTED_EDGE('',*,*,#900,.T.);
#1434=CYLINDRICAL_SURFACE('',#1750,12.7);
#1435=CYLINDRICAL_SURFACE('',#1753,4.826);
#1436=CYLINDRICAL_SURFACE('',#1756,76.1999999999999);
#1437=CYLINDRICAL_SURFACE('',#1759,4.826);
#1438=CYLINDRICAL_SURFACE('',#1762,8.88999999999999);
#1439=CYLINDRICAL_SURFACE('',#1801,4.826);
#1440=CYLINDRICAL_SURFACE('',#1803,27.0465001077289);
#1441=CYLINDRICAL_SURFACE('',#1804,76.2);
#1442=CYLINDRICAL_SURFACE('',#1805,27.0465001077289);
#1443=CYLINDRICAL_SURFACE('',#1807,4.826);
#1444=CYLINDRICAL_SURFACE('',#1809,27.0465001077289);
#1445=CYLINDRICAL_SURFACE('',#1810,76.1999999999999);
#1446=CYLINDRICAL_SURFACE('',#1811,27.0465001077289);
#1447=CYLINDRICAL_SURFACE('',#1814,27.0465001077289);
#1448=CYLINDRICAL_SURFACE('',#1815,27.0465001077289);
#1449=CYLINDRICAL_SURFACE('',#1818,27.0465001077289);
#1450=CYLINDRICAL_SURFACE('',#1819,76.1999999999999);
#1451=CYLINDRICAL_SURFACE('',#1820,27.0465001077289);
#1452=CYLINDRICAL_SURFACE('',#1822,4.826);
#1453=CYLINDRICAL_SURFACE('',#1824,27.0465001077289);
#1454=CYLINDRICAL_SURFACE('',#1825,76.1999999999999);
#1455=CYLINDRICAL_SURFACE('',#1826,27.0465001077289);
#1509=ADVANCED_FACE('',(#178),#1434,.F.);
#1510=ADVANCED_FACE('',(#179),#1435,.F.);
#1511=ADVANCED_FACE('',(#180),#1436,.F.);
#1512=ADVANCED_FACE('',(#181),#1437,.F.);
#1513=ADVANCED_FACE('',(#182),#1438,.F.);
#1514=ADVANCED_FACE('',(#183,#95),#111,.T.);
#1515=ADVANCED_FACE('',(#184,#96),#112,.F.);
#1516=ADVANCED_FACE('',(#185),#1439,.F.);
#1517=ADVANCED_FACE('',(#186),#113,.F.);
#1518=ADVANCED_FACE('',(#187),#1440,.T.);
#1519=ADVANCED_FACE('',(#188),#1441,.F.);
#1520=ADVANCED_FACE('',(#189),#1442,.T.);
#1521=ADVANCED_FACE('',(#190),#114,.F.);
#1522=ADVANCED_FACE('',(#191),#1443,.F.);
#1523=ADVANCED_FACE('',(#192),#115,.F.);
#1524=ADVANCED_FACE('',(#193),#1444,.T.);
#1525=ADVANCED_FACE('',(#194),#1445,.F.);
#1526=ADVANCED_FACE('',(#195),#1446,.T.);
#1527=ADVANCED_FACE('',(#196),#116,.F.);
#1528=ADVANCED_FACE('',(#197),#117,.F.);
#1529=ADVANCED_FACE('',(#198),#1447,.T.);
#1530=ADVANCED_FACE('',(#199),#1448,.T.);
#1531=ADVANCED_FACE('',(#200),#118,.F.);
#1532=ADVANCED_FACE('',(#201),#119,.F.);
#1533=ADVANCED_FACE('',(#202),#1449,.T.);
#1534=ADVANCED_FACE('',(#203),#1450,.F.);
#1535=ADVANCED_FACE('',(#204),#1451,.T.);
#1536=ADVANCED_FACE('',(#205),#120,.F.);
#1537=ADVANCED_FACE('',(#206),#1452,.F.);
#1538=ADVANCED_FACE('',(#207),#121,.F.);
#1539=ADVANCED_FACE('',(#208),#1453,.T.);
#1540=ADVANCED_FACE('',(#209),#1454,.F.);
#1541=ADVANCED_FACE('',(#210),#1455,.T.);
#1542=ADVANCED_FACE('',(#211),#122,.F.);
#1543=ADVANCED_FACE('',(#212,#97),#123,.T.);
#1551=CLOSED_SHELL('',(#1509,#1510,#1511,#1512,#1513,#1514,#1515,#1516,
#1517,#1518,#1519,#1520,#1521,#1522,#1523,#1524,#1525,#1526,#1527,#1528,
#1529,#1530,#1531,#1532,#1533,#1534,#1535,#1536,#1537,#1538,#1539,#1540,
#1541,#1542,#1543));
#1749=AXIS2_PLACEMENT_3D('',#2614,#2139,#2140);
#1750=AXIS2_PLACEMENT_3D('',#2615,#2141,#2142);
#1751=AXIS2_PLACEMENT_3D('',#2617,#2143,#2144);
#1752=AXIS2_PLACEMENT_3D('',#2620,#2146,#2147);
#1753=AXIS2_PLACEMENT_3D('',#2621,#2148,#2149);
#1754=AXIS2_PLACEMENT_3D('',#2624,#2150,#2151);
#1755=AXIS2_PLACEMENT_3D('',#2628,#2153,#2154);
#1756=AXIS2_PLACEMENT_3D('',#2630,#2156,#2157);
#1757=AXIS2_PLACEMENT_3D('',#2633,#2158,#2159);
#1758=AXIS2_PLACEMENT_3D('',#2637,#2161,#2162);
#1759=AXIS2_PLACEMENT_3D('',#2639,#2164,#2165);
#1760=AXIS2_PLACEMENT_3D('',#2642,#2166,#2167);
#1761=AXIS2_PLACEMENT_3D('',#2646,#2169,#2170);
#1762=AXIS2_PLACEMENT_3D('',#2648,#2172,#2173);
#1763=AXIS2_PLACEMENT_3D('',#2650,#2174,#2175);
#1764=AXIS2_PLACEMENT_3D('',#2653,#2177,#2178);
#1765=AXIS2_PLACEMENT_3D('',#2654,#2179,#2180);
#1766=AXIS2_PLACEMENT_3D('',#2657,#2181,#2182);
#1767=AXIS2_PLACEMENT_3D('',#2661,#2184,#2185);
#1768=AXIS2_PLACEMENT_3D('',#2663,#2186,#2187);
#1769=AXIS2_PLACEMENT_3D('',#2665,#2188,#2189);
#1770=AXIS2_PLACEMENT_3D('',#2669,#2191,#2192);
#1771=AXIS2_PLACEMENT_3D('',#2673,#2194,#2195);
#1772=AXIS2_PLACEMENT_3D('',#2675,#2196,#2197);
#1773=AXIS2_PLACEMENT_3D('',#2677,#2198,#2199);
#1774=AXIS2_PLACEMENT_3D('',#2681,#2202,#2203);
#1775=AXIS2_PLACEMENT_3D('',#2683,#2204,#2205);
#1776=AXIS2_PLACEMENT_3D('',#2688,#2208,#2209);
#1777=AXIS2_PLACEMENT_3D('',#2690,#2210,#2211);
#1778=AXIS2_PLACEMENT_3D('',#2692,#2212,#2213);
#1779=AXIS2_PLACEMENT_3D('',#2696,#2215,#2216);
#1780=AXIS2_PLACEMENT_3D('',#2700,#2218,#2219);
#1781=AXIS2_PLACEMENT_3D('',#2702,#2220,#2221);
#1782=AXIS2_PLACEMENT_3D('',#2704,#2222,#2223);
#1783=AXIS2_PLACEMENT_3D('',#2706,#2225,#2226);
#1784=AXIS2_PLACEMENT_3D('',#2709,#2227,#2228);
#1785=AXIS2_PLACEMENT_3D('',#2713,#2230,#2231);
#1786=AXIS2_PLACEMENT_3D('',#2715,#2232,#2233);
#1787=AXIS2_PLACEMENT_3D('',#2717,#2234,#2235);
#1788=AXIS2_PLACEMENT_3D('',#2721,#2237,#2238);
#1789=AXIS2_PLACEMENT_3D('',#2725,#2240,#2241);
#1790=AXIS2_PLACEMENT_3D('',#2727,#2242,#2243);
#1791=AXIS2_PLACEMENT_3D('',#2729,#2244,#2245);
#1792=AXIS2_PLACEMENT_3D('',#2733,#2248,#2249);
#1793=AXIS2_PLACEMENT_3D('',#2735,#2250,#2251);
#1794=AXIS2_PLACEMENT_3D('',#2740,#2254,#2255);
#1795=AXIS2_PLACEMENT_3D('',#2742,#2256,#2257);
#1796=AXIS2_PLACEMENT_3D('',#2744,#2258,#2259);
#1797=AXIS2_PLACEMENT_3D('',#2748,#2261,#2262);
#1798=AXIS2_PLACEMENT_3D('',#2752,#2264,#2265);
#1799=AXIS2_PLACEMENT_3D('',#2754,#2266,#2267);
#1800=AXIS2_PLACEMENT_3D('',#2756,#2268,#2269);
#1801=AXIS2_PLACEMENT_3D('',#2758,#2271,#2272);
#1802=AXIS2_PLACEMENT_3D('',#2761,#2275,#2276);
#1803=AXIS2_PLACEMENT_3D('',#2763,#2278,#2279);
#1804=AXIS2_PLACEMENT_3D('',#2765,#2281,#2282);
#1805=AXIS2_PLACEMENT_3D('',#2767,#2284,#2285);
#1806=AXIS2_PLACEMENT_3D('',#2769,#2287,#2288);
#1807=AXIS2_PLACEMENT_3D('',#2771,#2290,#2291);
#1808=AXIS2_PLACEMENT_3D('',#2773,#2293,#2294);
#1809=AXIS2_PLACEMENT_3D('',#2775,#2296,#2297);
#1810=AXIS2_PLACEMENT_3D('',#2777,#2299,#2300);
#1811=AXIS2_PLACEMENT_3D('',#2779,#2302,#2303);
#1812=AXIS2_PLACEMENT_3D('',#2781,#2305,#2306);
#1813=AXIS2_PLACEMENT_3D('',#2782,#2307,#2308);
#1814=AXIS2_PLACEMENT_3D('',#2784,#2310,#2311);
#1815=AXIS2_PLACEMENT_3D('',#2785,#2312,#2313);
#1816=AXIS2_PLACEMENT_3D('',#2787,#2315,#2316);
#1817=AXIS2_PLACEMENT_3D('',#2788,#2317,#2318);
#1818=AXIS2_PLACEMENT_3D('',#2790,#2320,#2321);
#1819=AXIS2_PLACEMENT_3D('',#2792,#2323,#2324);
#1820=AXIS2_PLACEMENT_3D('',#2794,#2326,#2327);
#1821=AXIS2_PLACEMENT_3D('',#2796,#2329,#2330);
#1822=AXIS2_PLACEMENT_3D('',#2798,#2332,#2333);
#1823=AXIS2_PLACEMENT_3D('',#2800,#2335,#2336);
#1824=AXIS2_PLACEMENT_3D('',#2802,#2338,#2339);
#1825=AXIS2_PLACEMENT_3D('',#2804,#2341,#2342);
#1826=AXIS2_PLACEMENT_3D('',#2806,#2344,#2345);
#1827=AXIS2_PLACEMENT_3D('',#2808,#2347,#2348);
#1828=AXIS2_PLACEMENT_3D('',#2809,#2349,#2350);
#2139=DIRECTION('axis',(0.,0.,1.));
#2140=DIRECTION('refdir',(1.,0.,0.));
#2141=DIRECTION('center_axis',(2.61947219093537E-16,1.,-5.05688216913818E-17));
#2142=DIRECTION('ref_axis',(-1.10981324742611E-16,5.05688216913819E-17,
1.));
#2143=DIRECTION('center_axis',(2.61947219093537E-16,1.,-5.05688216913818E-17));
#2144=DIRECTION('ref_axis',(-1.10981324742611E-16,5.05688216913819E-17,
1.));
#2145=DIRECTION('',(2.61947219093537E-16,1.,-5.05688216913818E-17));
#2146=DIRECTION('center_axis',(2.61947219093537E-16,1.,-5.05688216913818E-17));
#2147=DIRECTION('ref_axis',(-1.10981324742611E-16,5.05688216913819E-17,
1.));
#2148=DIRECTION('center_axis',(-2.61947219093537E-16,-1.,5.05688216913818E-17));
#2149=DIRECTION('ref_axis',(-1.32463622148944E-32,-5.05688216913818E-17,
-1.));
#2150=DIRECTION('center_axis',(-2.61947219093537E-16,-1.,5.05688216913818E-17));
#2151=DIRECTION('ref_axis',(1.32463622148944E-32,5.05688216913818E-17,1.));
#2152=DIRECTION('',(-2.61947219093537E-16,-1.,5.05688216913818E-17));
#2153=DIRECTION('center_axis',(-2.61947219093537E-16,-1.,5.05688216913818E-17));
#2154=DIRECTION('ref_axis',(2.64927244297885E-32,5.05688216913818E-17,1.));
#2155=DIRECTION('',(-2.61947219093537E-16,-1.,5.05688216913818E-17));
#2156=DIRECTION('center_axis',(-2.61947219093537E-16,-1.,5.05688216913818E-17));
#2157=DIRECTION('ref_axis',(1.10981324742611E-16,-5.05688216913819E-17,
-1.));
#2158=DIRECTION('center_axis',(-2.61947219093537E-16,-1.,5.05688216913818E-17));
#2159=DIRECTION('ref_axis',(1.10981324742611E-16,-5.05688216913819E-17,
-1.));
#2160=DIRECTION('',(-2.61947219093537E-16,-1.,5.05688216913818E-17));
#2161=DIRECTION('center_axis',(-2.61947219093537E-16,-1.,5.05688216913818E-17));
#2162=DIRECTION('ref_axis',(1.10981324742611E-16,-5.05688216913819E-17,
-1.));
#2163=DIRECTION('',(-2.61947219093537E-16,-1.,5.05688216913818E-17));
#2164=DIRECTION('center_axis',(-2.61947219093537E-16,-1.,5.05688216913818E-17));
#2165=DIRECTION('ref_axis',(-1.32463622148944E-32,-5.05688216913818E-17,
-1.));
#2166=DIRECTION('center_axis',(-2.61947219093537E-16,-1.,5.05688216913818E-17));
#2167=DIRECTION('ref_axis',(1.32463622148944E-32,5.05688216913818E-17,1.));
#2168=DIRECTION('',(-2.61947219093537E-16,-1.,5.05688216913818E-17));
#2169=DIRECTION('center_axis',(-2.61947219093537E-16,-1.,5.05688216913818E-17));
#2170=DIRECTION('ref_axis',(2.64927244297889E-32,5.05688216913818E-17,1.));
#2171=DIRECTION('',(-2.61947219093537E-16,-1.,5.05688216913818E-17));
#2172=DIRECTION('center_axis',(-2.61947219093537E-16,-1.,5.05688216913818E-17));
#2173=DIRECTION('ref_axis',(1.09761749745439E-16,-5.05688216913819E-17,
-1.));
#2174=DIRECTION('center_axis',(-2.61947219093537E-16,-1.,5.05688216913818E-17));
#2175=DIRECTION('ref_axis',(-1.88729230812297E-15,5.05688216913823E-17,
1.));
#2176=DIRECTION('',(-2.61947219093537E-16,-1.,5.05688216913819E-17));
#2177=DIRECTION('center_axis',(-2.61947219093537E-16,-1.,5.05688216913818E-17));
#2178=DIRECTION('ref_axis',(1.09761749745439E-16,-5.05688216913819E-17,
-1.));
#2179=DIRECTION('center_axis',(2.61947219093537E-16,1.,5.0568821691382E-17));
#2180=DIRECTION('ref_axis',(-1.11022302462516E-16,-5.0568821691382E-17,
1.));
#2181=DIRECTION('center_axis',(-2.61947219093537E-16,-1.,5.05688216913818E-17));
#2182=DIRECTION('ref_axis',(-1.12329276055274E-16,5.05688216913819E-17,
1.));
#2183=DIRECTION('',(1.11022302462516E-16,5.0568821691382E-17,-1.));
#2184=DIRECTION('center_axis',(2.61947219093537E-16,1.,-5.05688216913818E-17));
#2185=DIRECTION('ref_axis',(-1.12242473919644E-16,5.05688216913819E-17,
1.));
#2186=DIRECTION('center_axis',(-2.61947219093537E-16,-1.,5.05688216913818E-17));
#2187=DIRECTION('ref_axis',(-1.82123199577618E-16,5.05688216913819E-17,
1.));
#2188=DIRECTION('center_axis',(2.61947219093537E-16,1.,-5.05688216913818E-17));
#2189=DIRECTION('ref_axis',(-3.00472787334257E-32,-5.05688216913818E-17,
-1.));
#2190=DIRECTION('',(0.951056516295154,2.33499984356149E-16,0.309016994374947));
#2191=DIRECTION('center_axis',(-2.61947219093537E-16,-1.,5.05688216913818E-17));
#2192=DIRECTION('ref_axis',(1.32463622148944E-32,5.05688216913818E-17,1.));
#2193=DIRECTION('',(-0.951056516295154,-2.33499984356149E-16,-0.309016994374947));
#2194=DIRECTION('center_axis',(2.61947219093537E-16,1.,-5.05688216913818E-17));
#2195=DIRECTION('ref_axis',(3.00472787334257E-32,5.05688216913818E-17,1.));
#2196=DIRECTION('center_axis',(-2.61947219093537E-16,-1.,5.05688216913818E-17));
#2197=DIRECTION('ref_axis',(-2.5173028630338E-32,-5.05688216913818E-17,
-1.));
#2198=DIRECTION('center_axis',(2.61947219093537E-16,1.,-5.05688216913818E-17));
#2199=DIRECTION('ref_axis',(-3.00472787334257E-32,-5.05688216913818E-17,
-1.));
#2200=DIRECTION('',(0.587785252292473,1.94879748396051E-16,-0.809016994374948));
#2201=DIRECTION('',(-0.587785252292473,-1.94879748396051E-16,0.809016994374947));
#2202=DIRECTION('center_axis',(2.61947219093537E-16,1.,-5.05688216913818E-17));
#2203=DIRECTION('ref_axis',(3.00472787334257E-32,5.05688216913818E-17,1.));
#2204=DIRECTION('center_axis',(2.61947219093537E-16,1.,-5.05688216913818E-17));
#2205=DIRECTION('ref_axis',(-3.00472787334257E-32,-5.05688216913818E-17,
-1.));
#2206=DIRECTION('',(-0.587785252292473,-1.13057676128363E-16,-0.809016994374947));
#2207=DIRECTION('',(0.587785252292473,1.13057676128363E-16,0.809016994374947));
#2208=DIRECTION('center_axis',(2.61947219093537E-16,1.,-5.05688216913818E-17));
#2209=DIRECTION('ref_axis',(3.00472787334257E-32,5.05688216913818E-17,1.));
#2210=DIRECTION('center_axis',(-2.61947219093537E-16,-1.,5.05688216913818E-17));
#2211=DIRECTION('ref_axis',(-2.5173028630338E-32,-5.05688216913818E-17,
-1.));
#2212=DIRECTION('center_axis',(2.61947219093537E-16,1.,-5.05688216913818E-17));
#2213=DIRECTION('ref_axis',(-3.00472787334257E-32,-5.05688216913818E-17,
-1.));
#2214=DIRECTION('',(-0.951056516295154,-2.64753234932456E-16,0.309016994374947));
#2215=DIRECTION('center_axis',(-2.61947219093537E-16,-1.,5.05688216913818E-17));
#2216=DIRECTION('ref_axis',(1.32463622148944E-32,5.05688216913818E-17,1.));
#2217=DIRECTION('',(0.951056516295154,2.64753234932456E-16,-0.309016994374947));
#2218=DIRECTION('center_axis',(2.61947219093537E-16,1.,-5.05688216913818E-17));
#2219=DIRECTION('ref_axis',(3.00472787334257E-32,5.05688216913818E-17,1.));
#2220=DIRECTION('center_axis',(-2.61947219093537E-16,-1.,5.05688216913818E-17));
#2221=DIRECTION('ref_axis',(1.82123199577618E-16,-5.05688216913819E-17,
-1.));
#2222=DIRECTION('center_axis',(2.61947219093537E-16,1.,-5.05688216913818E-17));
#2223=DIRECTION('ref_axis',(1.12242473919644E-16,-5.05688216913819E-17,
-1.));
#2224=DIRECTION('',(-1.11022302462516E-16,-5.0568821691382E-17,1.));
#2225=DIRECTION('center_axis',(2.61947219093537E-16,1.,5.0568821691382E-17));
#2226=DIRECTION('ref_axis',(-1.11022302462516E-16,-5.0568821691382E-17,
1.));
#2227=DIRECTION('center_axis',(-2.61947219093537E-16,-1.,5.05688216913818E-17));
#2228=DIRECTION('ref_axis',(-1.12329276055274E-16,5.05688216913819E-17,
1.));
#2229=DIRECTION('',(-1.11022302462516E-16,-5.0568821691382E-17,1.));
#2230=DIRECTION('center_axis',(2.61947219093537E-16,1.,-5.05688216913818E-17));
#2231=DIRECTION('ref_axis',(1.12242473919644E-16,-5.05688216913819E-17,
-1.));
#2232=DIRECTION('center_axis',(-2.61947219093537E-16,-1.,5.05688216913818E-17));
#2233=DIRECTION('ref_axis',(1.82123199577618E-16,-5.05688216913819E-17,
-1.));
#2234=DIRECTION('center_axis',(2.61947219093537E-16,1.,-5.05688216913818E-17));
#2235=DIRECTION('ref_axis',(2.64927244297889E-32,5.05688216913818E-17,1.));
#2236=DIRECTION('',(0.951056516295154,2.64753234932456E-16,-0.309016994374947));
#2237=DIRECTION('center_axis',(-2.61947219093537E-16,-1.,5.05688216913818E-17));
#2238=DIRECTION('ref_axis',(2.64927244297892E-32,5.05688216913818E-17,1.));
#2239=DIRECTION('',(-0.951056516295154,-2.64753234932456E-16,0.309016994374947));
#2240=DIRECTION('center_axis',(2.61947219093537E-16,1.,-5.05688216913818E-17));
#2241=DIRECTION('ref_axis',(-2.64927244297889E-32,-5.05688216913818E-17,
-1.));
#2242=DIRECTION('center_axis',(-2.61947219093537E-16,-1.,5.05688216913818E-17));
#2243=DIRECTION('ref_axis',(-2.64927244297889E-32,-5.05688216913818E-17,
-1.));
#2244=DIRECTION('center_axis',(2.61947219093537E-16,1.,-5.05688216913818E-17));
#2245=DIRECTION('ref_axis',(2.64927244297889E-32,5.05688216913818E-17,1.));
#2246=DIRECTION('',(0.587785252292473,1.13057676128363E-16,0.809016994374947));
#2247=DIRECTION('',(-0.587785252292473,-1.13057676128363E-16,-0.809016994374947));
#2248=DIRECTION('center_axis',(2.61947219093537E-16,1.,-5.05688216913818E-17));
#2249=DIRECTION('ref_axis',(-2.64927244297889E-32,-5.05688216913818E-17,
-1.));
#2250=DIRECTION('center_axis',(2.61947219093537E-16,1.,-5.05688216913818E-17));
#2251=DIRECTION('ref_axis',(2.64927244297889E-32,5.05688216913818E-17,1.));
#2252=DIRECTION('',(-0.587785252292473,-1.94879748396051E-16,0.809016994374947));
#2253=DIRECTION('',(0.587785252292473,1.94879748396051E-16,-0.809016994374948));
#2254=DIRECTION('center_axis',(2.61947219093537E-16,1.,-5.05688216913818E-17));
#2255=DIRECTION('ref_axis',(-2.64927244297889E-32,-5.05688216913818E-17,
-1.));
#2256=DIRECTION('center_axis',(-2.61947219093537E-16,-1.,5.05688216913818E-17));
#2257=DIRECTION('ref_axis',(-2.64927244297889E-32,-5.05688216913818E-17,
-1.));
#2258=DIRECTION('center_axis',(2.61947219093537E-16,1.,-5.05688216913818E-17));
#2259=DIRECTION('ref_axis',(2.64927244297889E-32,5.05688216913818E-17,1.));
#2260=DIRECTION('',(-0.951056516295154,-2.33499984356149E-16,-0.309016994374947));
#2261=DIRECTION('center_axis',(-2.61947219093537E-16,-1.,5.05688216913818E-17));
#2262=DIRECTION('ref_axis',(2.64927244297889E-32,5.05688216913818E-17,1.));
#2263=DIRECTION('',(0.951056516295154,2.33499984356149E-16,0.309016994374947));
#2264=DIRECTION('center_axis',(2.61947219093537E-16,1.,-5.05688216913818E-17));
#2265=DIRECTION('ref_axis',(-2.64927244297889E-32,-5.05688216913818E-17,
-1.));
#2266=DIRECTION('center_axis',(-2.61947219093537E-16,-1.,5.05688216913818E-17));
#2267=DIRECTION('ref_axis',(-1.82123199577618E-16,5.05688216913819E-17,
1.));
#2268=DIRECTION('center_axis',(2.61947219093537E-16,1.,-5.05688216913818E-17));
#2269=DIRECTION('ref_axis',(-1.12242473919644E-16,5.05688216913819E-17,
1.));
#2270=DIRECTION('',(1.11022302462516E-16,5.0568821691382E-17,-1.));
#2271=DIRECTION('center_axis',(-2.61947219093537E-16,-1.,5.05688216913818E-17));
#2272=DIRECTION('ref_axis',(4.6195413228266E-14,5.05688216913697E-17,1.));
#2273=DIRECTION('',(-2.61947219093537E-16,-1.,5.05688216913818E-17));
#2274=DIRECTION('',(-2.61947219093537E-16,-1.,5.05688216913818E-17));
#2275=DIRECTION('center_axis',(-1.,-2.61947219093537E-16,-1.11022302462516E-16));
#2276=DIRECTION('ref_axis',(-1.11022302462516E-16,-5.0568821691382E-17,
1.));
#2277=DIRECTION('',(-2.61947219093537E-16,-1.,5.05688216913818E-17));
#2278=DIRECTION('center_axis',(-2.61947219093537E-16,-1.,5.05688216913818E-17));
#2279=DIRECTION('ref_axis',(1.12242473919644E-16,-5.05688216913819E-17,
-1.));
#2280=DIRECTION('',(-2.61947219093537E-16,-1.,5.05688216913818E-17));
#2281=DIRECTION('center_axis',(-2.61947219093537E-16,-1.,5.05688216913818E-17));
#2282=DIRECTION('ref_axis',(1.82123199577618E-16,-5.05688216913819E-17,
-1.));
#2283=DIRECTION('',(-2.61947219093537E-16,-1.,5.05688216913818E-17));
#2284=DIRECTION('center_axis',(-2.61947219093537E-16,-1.,5.05688216913818E-17));
#2285=DIRECTION('ref_axis',(-3.00472787334257E-32,-5.05688216913818E-17,
-1.));
#2286=DIRECTION('',(-2.61947219093537E-16,-1.,5.05688216913818E-17));
#2287=DIRECTION('center_axis',(0.309016994374947,1.29039949720116E-16,-0.951056516295154));
#2288=DIRECTION('ref_axis',(-0.951056516295154,-2.33499984356149E-16,-0.309016994374947));
#2289=DIRECTION('',(-2.61947219093537E-16,-1.,5.05688216913818E-17));
#2290=DIRECTION('center_axis',(-2.61947219093537E-16,-1.,5.05688216913818E-17));
#2291=DIRECTION('ref_axis',(0.95105651629515,-2.33499984356148E-16,0.309016994374957));
#2292=DIRECTION('',(-2.61947219093537E-16,-1.,5.05688216913818E-17));
#2293=DIRECTION('center_axis',(-0.309016994374947,-1.29039949720117E-16,
0.951056516295154));
#2294=DIRECTION('ref_axis',(0.951056516295154,2.33499984356149E-16,0.309016994374947));
#2295=DIRECTION('',(-2.61947219093537E-16,-1.,5.05688216913818E-17));
#2296=DIRECTION('center_axis',(-2.61947219093537E-16,-1.,5.05688216913818E-17));
#2297=DIRECTION('ref_axis',(-3.00472787334257E-32,-5.05688216913818E-17,
-1.));
#2298=DIRECTION('',(-2.61947219093537E-16,-1.,5.05688216913818E-17));
#2299=DIRECTION('center_axis',(-2.61947219093537E-16,-1.,5.05688216913818E-17));
#2300=DIRECTION('ref_axis',(-2.5173028630338E-32,-5.05688216913818E-17,
-1.));
#2301=DIRECTION('',(-2.61947219093537E-16,-1.,5.05688216913818E-17));
#2302=DIRECTION('center_axis',(-2.61947219093537E-16,-1.,5.05688216913818E-17));
#2303=DIRECTION('ref_axis',(-3.00472787334257E-32,-5.05688216913818E-17,
-1.));
#2304=DIRECTION('',(-2.61947219093537E-16,-1.,5.05688216913818E-17));
#2305=DIRECTION('center_axis',(-0.809016994374948,-1.82196144259928E-16,
-0.587785252292473));
#2306=DIRECTION('ref_axis',(-0.587785252292473,-1.94879748396051E-16,0.809016994374948));
#2307=DIRECTION('center_axis',(0.809016994374948,1.82196144259928E-16,0.587785252292473));
#2308=DIRECTION('ref_axis',(0.587785252292473,1.94879748396051E-16,-0.809016994374948));
#2309=DIRECTION('',(-2.61947219093537E-16,-1.,5.05688216913818E-17));
#2310=DIRECTION('center_axis',(-2.61947219093537E-16,-1.,5.05688216913818E-17));
#2311=DIRECTION('ref_axis',(-3.00472787334257E-32,-5.05688216913818E-17,
-1.));
#2312=DIRECTION('center_axis',(-2.61947219093537E-16,-1.,5.05688216913818E-17));
#2313=DIRECTION('ref_axis',(-3.00472787334257E-32,-5.05688216913818E-17,
-1.));
#2314=DIRECTION('',(-2.61947219093537E-16,-1.,5.05688216913818E-17));
#2315=DIRECTION('center_axis',(-0.809016994374947,-2.41643359491932E-16,
0.587785252292473));
#2316=DIRECTION('ref_axis',(0.587785252292473,1.13057676128362E-16,0.809016994374948));
#2317=DIRECTION('center_axis',(0.809016994374947,2.41643359491932E-16,-0.587785252292473));
#2318=DIRECTION('ref_axis',(-0.587785252292473,-1.13057676128362E-16,-0.809016994374947));
#2319=DIRECTION('',(-2.61947219093537E-16,-1.,5.05688216913818E-17));
#2320=DIRECTION('center_axis',(-2.61947219093537E-16,-1.,5.05688216913818E-17));
#2321=DIRECTION('ref_axis',(-3.00472787334257E-32,-5.05688216913818E-17,
-1.));
#2322=DIRECTION('',(-2.61947219093537E-16,-1.,5.05688216913818E-17));
#2323=DIRECTION('center_axis',(-2.61947219093537E-16,-1.,5.05688216913818E-17));
#2324=DIRECTION('ref_axis',(-2.5173028630338E-32,-5.05688216913818E-17,
-1.));
#2325=DIRECTION('',(-2.61947219093537E-16,-1.,5.05688216913818E-17));
#2326=DIRECTION('center_axis',(-2.61947219093537E-16,-1.,5.05688216913818E-17));
#2327=DIRECTION('ref_axis',(-3.00472787334257E-32,-5.05688216913818E-17,
-1.));
#2328=DIRECTION('',(-2.61947219093537E-16,-1.,5.05688216913818E-17));
#2329=DIRECTION('center_axis',(0.309016994374947,3.28523349382053E-17,0.951056516295154));
#2330=DIRECTION('ref_axis',(0.951056516295154,2.64753234932456E-16,-0.309016994374947));
#2331=DIRECTION('',(-2.61947219093537E-16,-1.,5.05688216913818E-17));
#2332=DIRECTION('center_axis',(-2.61947219093537E-16,-1.,5.05688216913818E-17));
#2333=DIRECTION('ref_axis',(-0.951056516295152,2.64753234932456E-16,0.309016994374953));
#2334=DIRECTION('',(-2.61947219093537E-16,-1.,5.05688216913818E-17));
#2335=DIRECTION('center_axis',(-0.309016994374947,-3.28523349382053E-17,
-0.951056516295154));
#2336=DIRECTION('ref_axis',(-0.951056516295154,-2.64753234932456E-16,0.309016994374947));
#2337=DIRECTION('',(-2.61947219093537E-16,-1.,5.05688216913818E-17));
#2338=DIRECTION('center_axis',(-2.61947219093537E-16,-1.,5.05688216913818E-17));
#2339=DIRECTION('ref_axis',(-3.00472787334257E-32,-5.05688216913818E-17,
-1.));
#2340=DIRECTION('',(-2.61947219093537E-16,-1.,5.05688216913818E-17));
#2341=DIRECTION('center_axis',(-2.61947219093537E-16,-1.,5.05688216913818E-17));
#2342=DIRECTION('ref_axis',(1.82123199577618E-16,-5.05688216913819E-17,
-1.));
#2343=DIRECTION('',(-2.61947219093537E-16,-1.,5.05688216913818E-17));
#2344=DIRECTION('center_axis',(-2.61947219093537E-16,-1.,5.05688216913818E-17));
#2345=DIRECTION('ref_axis',(1.12242473919644E-16,-5.05688216913819E-17,
-1.));
#2346=DIRECTION('',(-2.61947219093537E-16,-1.,5.05688216913818E-17));
#2347=DIRECTION('center_axis',(1.,2.61947219093537E-16,1.11022302462516E-16));
#2348=DIRECTION('ref_axis',(1.11022302462516E-16,5.0568821691382E-17,-1.));
#2349=DIRECTION('center_axis',(2.61947219093537E-16,1.,5.0568821691382E-17));
#2350=DIRECTION('ref_axis',(-1.11022302462516E-16,-5.0568821691382E-17,
1.));
#2614=CARTESIAN_POINT('',(0.,0.,0.));
#2615=CARTESIAN_POINT('Origin',(0.196389981728107,9.52499999999995,14.3245422672531));
#2616=CARTESIAN_POINT('',(0.196389981728107,9.52499999999995,1.62454226725312));
#2617=CARTESIAN_POINT('Origin',(0.196389981728107,9.52499999999995,14.3245422672531));
#2618=CARTESIAN_POINT('',(0.196389981728107,12.6999999999999,1.62454226725311));
#2619=CARTESIAN_POINT('',(0.196389981728107,9.52499999999995,1.62454226725312));
#2620=CARTESIAN_POINT('Origin',(0.196389981728107,12.6999999999999,14.3245422672531));
#2621=CARTESIAN_POINT('Origin',(29.1600960736921,12.7000000000002,54.1896636820751));
#2622=CARTESIAN_POINT('',(25.2557800588381,12.7,57.0263153096353));
#2623=CARTESIAN_POINT('',(33.0644120885452,12.7000000000002,51.3530120545092));
#2624=CARTESIAN_POINT('Origin',(29.1600960736921,12.7000000000002,54.1896636820751));
#2625=CARTESIAN_POINT('',(25.2557800588381,0.,57.0263153096353));
#2626=CARTESIAN_POINT('',(25.2557800588381,12.7,57.0263153096353));
#2627=CARTESIAN_POINT('',(33.0644120885454,1.66533453693773E-13,51.3530120545087));
#2628=CARTESIAN_POINT('Origin',(29.1600960736921,1.66533453693773E-13,54.1896636820751));
#2629=CARTESIAN_POINT('',(33.0644120885452,12.7000000000002,51.3530120545092));
#2630=CARTESIAN_POINT('Origin',(0.196389981727885,12.6999999999999,154.439874761711));
#2631=CARTESIAN_POINT('',(-44.54372429145,12.6999999999999,92.7571204877404));
#2632=CARTESIAN_POINT('',(44.9365042549055,12.7000000000001,92.7571204877395));
#2633=CARTESIAN_POINT('Origin',(0.196389981727885,12.6999999999999,154.439874761711));
#2634=CARTESIAN_POINT('',(-44.54372429145,-5.55111512312578E-14,92.7571204877404));
#2635=CARTESIAN_POINT('',(-44.54372429145,12.6999999999999,92.7571204877404));
#2636=CARTESIAN_POINT('',(44.9365042549055,1.11022302462516E-13,92.7571204877395));
#2637=CARTESIAN_POINT('Origin',(0.196389981727996,-5.55111512312578E-14,
154.439874761711));
#2638=CARTESIAN_POINT('',(44.9365042549055,12.7000000000001,92.7571204877395));
#2639=CARTESIAN_POINT('Origin',(-28.767316110236,12.6999999999999,54.1896636820724));
#2640=CARTESIAN_POINT('',(-32.6716321250896,12.7,51.35301205451));
#2641=CARTESIAN_POINT('',(-24.8630000953821,12.7000000000001,57.0263153096384));
#2642=CARTESIAN_POINT('Origin',(-28.767316110236,12.6999999999999,54.1896636820724));
#2643=CARTESIAN_POINT('',(-32.6716321250895,0.,51.3530120545105));
#2644=CARTESIAN_POINT('',(-32.6716321250896,12.7,51.35301205451));
#2645=CARTESIAN_POINT('',(-24.8630000953821,1.11022302462516E-13,57.0263153096384));
#2646=CARTESIAN_POINT('Origin',(-28.767316110236,0.,54.1896636820724));
#2647=CARTESIAN_POINT('',(-24.8630000953821,12.7000000000001,57.0263153096384));
#2648=CARTESIAN_POINT('Origin',(0.196389981728107,59.182,14.3245422672531));
#2649=CARTESIAN_POINT('',(0.196389981728092,9.52499999999995,23.2145422672531));
#2650=CARTESIAN_POINT('Origin',(0.196389981728107,9.52499999999995,14.3245422672531));
#2651=CARTESIAN_POINT('',(0.196389981728089,-6.21724893790088E-14,23.2145422672531));
#2652=CARTESIAN_POINT('',(0.196389981728105,59.182,23.2145422672531));
#2653=CARTESIAN_POINT('Origin',(0.196389981728107,-5.55111512312578E-14,
14.3245422672531));
#2654=CARTESIAN_POINT('Origin',(0.196389981728107,12.7,-34.9514577327463));
#2655=CARTESIAN_POINT('',(5.02238998172821,12.7,-34.9514577327463));
#2656=CARTESIAN_POINT('',(-4.62961001827178,12.7,-34.9514577327459));
#2657=CARTESIAN_POINT('Origin',(0.196389981728107,12.7,-34.9514577327463));
#2658=CARTESIAN_POINT('',(-4.62961001827222,12.7000000000002,-76.5025437375311));
#2659=CARTESIAN_POINT('',(-4.62961001827178,12.7,-34.9514577327459));
#2660=CARTESIAN_POINT('',(-9.70961001827242,12.7000000000001,-75.4263257814172));
#2661=CARTESIAN_POINT('Origin',(-1.59000334476855,12.7000000000001,-49.6273886803462));
#2662=CARTESIAN_POINT('',(-82.1006355728287,12.6999999999999,-22.8311670701098));
#2663=CARTESIAN_POINT('Origin',(-82.1613360785705,12.6999999999999,-99.0311428932596));
#2664=CARTESIAN_POINT('',(-84.6939860043709,12.6999999999999,-18.332369605421));
#2665=CARTESIAN_POINT('Origin',(-60.07348477912,12.7000000000001,-7.13665223247828));
#2666=CARTESIAN_POINT('',(-45.1765549003784,12.7,-5.4923778952074));
#2667=CARTESIAN_POINT('',(-45.1765549003784,12.7,-5.4923778952074));
#2668=CARTESIAN_POINT('',(-48.1591869300858,12.7,3.68721960007434));
#2669=CARTESIAN_POINT('Origin',(-46.6678709152318,12.7,-0.902579147566751));
#2670=CARTESIAN_POINT('',(-87.6766180340772,12.6999999999999,-9.15277211013876));
#2671=CARTESIAN_POINT('',(-48.1591869300858,12.7,3.68721960007434));
#2672=CARTESIAN_POINT('',(-88.2228802653845,12.6999999999999,-3.98883536926853));
#2673=CARTESIAN_POINT('Origin',(-61.17753657217,12.7000000000001,-3.73873020481819));
#2674=CARTESIAN_POINT('',(-60.5719689840063,12.7000000000001,81.1119190693219));
#2675=CARTESIAN_POINT('Origin',(-133.061210019987,12.7,57.6225611805379));
#2676=CARTESIAN_POINT('',(-57.0947476954385,12.7000000000001,84.9685467671164));
#2677=CARTESIAN_POINT('Origin',(-38.8388344446712,12.7000000000001,65.0127255748467));
#2678=CARTESIAN_POINT('',(-32.6716321250896,12.7,51.35301205451));
#2679=CARTESIAN_POINT('',(-49.2861156657315,12.7,90.6418500222435));
#2680=CARTESIAN_POINT('',(-24.8630000953821,12.7000000000001,57.0263153096384));
#2681=CARTESIAN_POINT('Origin',(-35.9483893251246,12.7000000000001,67.1127568790628));
#2682=CARTESIAN_POINT('',(49.6788956291876,12.7000000000001,90.6418500222421));
#2683=CARTESIAN_POINT('Origin',(36.3411692885806,12.7000000000002,67.1127568790633));
#2684=CARTESIAN_POINT('',(25.2557800588381,12.7,57.0263153096353));
#2685=CARTESIAN_POINT('',(57.4875276588944,12.7000000000001,84.9685467671164));
#2686=CARTESIAN_POINT('',(33.0644120885452,12.7000000000002,51.3530120545092));
#2687=CARTESIAN_POINT('',(60.964748947462,12.7000000000002,81.1119190693224));
#2688=CARTESIAN_POINT('Origin',(39.2316144081271,12.7000000000002,65.0127255748485));
#2689=CARTESIAN_POINT('',(88.61566022884,12.7,-3.98883536926897));
#2690=CARTESIAN_POINT('Origin',(133.453989983443,12.7,57.6225611805374));
#2691=CARTESIAN_POINT('',(88.0693979975334,12.7,-9.15277211014009));
#2692=CARTESIAN_POINT('Origin',(61.5703165356259,12.7000000000001,-3.73873020481819));
#2693=CARTESIAN_POINT('',(48.5519668935416,12.7000000000002,3.6872196000739));
#2694=CARTESIAN_POINT('',(48.5519668935416,12.7000000000002,3.6872196000739));
#2695=CARTESIAN_POINT('',(45.5693348638345,12.7000000000002,-5.49237789520696));
#2696=CARTESIAN_POINT('Origin',(47.0606508786874,12.7000000000001,-0.902579147566307));
#2697=CARTESIAN_POINT('',(85.0867659678262,12.7000000000001,-18.3323696054205));
#2698=CARTESIAN_POINT('',(45.5693348638345,12.7000000000002,-5.49237789520696));
#2699=CARTESIAN_POINT('',(82.4934155362843,12.7000000000002,-22.831167070108));
#2700=CARTESIAN_POINT('Origin',(60.4662647425757,12.7000000000001,-7.13665223247784));
#2701=CARTESIAN_POINT('',(10.1023899817279,12.7000000000002,-75.4263257814172));
#2702=CARTESIAN_POINT('Origin',(82.5541160420259,12.7,-99.0311428932582));
#2703=CARTESIAN_POINT('',(5.02238998172799,12.7000000000001,-76.5025437375311));
#2704=CARTESIAN_POINT('Origin',(1.98278330822388,12.7000000000001,-49.6273886803467));
#2705=CARTESIAN_POINT('',(5.02238998172821,12.7,-34.9514577327463));
#2706=CARTESIAN_POINT('Origin',(0.196389981728218,0.,-34.9514577327463));
#2707=CARTESIAN_POINT('',(5.02238998172821,-5.55111512312578E-14,-34.9514577327463));
#2708=CARTESIAN_POINT('',(-4.62961001827178,0.,-34.9514577327459));
#2709=CARTESIAN_POINT('Origin',(0.196389981728218,0.,-34.9514577327463));
#2710=CARTESIAN_POINT('',(5.02238998172799,1.11022302462516E-13,-76.5025437375311));
#2711=CARTESIAN_POINT('',(5.02238998172821,-5.55111512312578E-14,-34.9514577327463));
#2712=CARTESIAN_POINT('',(10.1023899817279,1.66533453693773E-13,-75.4263257814172));
#2713=CARTESIAN_POINT('Origin',(1.98278330822388,1.11022302462516E-13,-49.6273886803467));
#2714=CARTESIAN_POINT('',(82.4934155362843,1.66533453693773E-13,-22.831167070108));
#2715=CARTESIAN_POINT('Origin',(82.5541160420259,0.,-99.0311428932586));
#2716=CARTESIAN_POINT('',(85.0867659678262,0.,-18.3323696054205));
#2717=CARTESIAN_POINT('Origin',(60.4662647425757,1.11022302462516E-13,-7.13665223247784));
#2718=CARTESIAN_POINT('',(45.5693348638345,1.66533453693773E-13,-5.49237789520696));
#2719=CARTESIAN_POINT('',(45.5693348638345,1.66533453693773E-13,-5.49237789520696));
#2720=CARTESIAN_POINT('',(48.5519668935416,1.66533453693773E-13,3.6872196000739));
#2721=CARTESIAN_POINT('Origin',(47.0606508786874,1.11022302462516E-13,-0.902579147566307));
#2722=CARTESIAN_POINT('',(88.0693979975334,0.,-9.15277211014009));
#2723=CARTESIAN_POINT('',(48.5519668935416,1.66533453693773E-13,3.6872196000739));
#2724=CARTESIAN_POINT('',(88.61566022884,0.,-3.98883536926897));
#2725=CARTESIAN_POINT('Origin',(61.5703165356259,1.11022302462516E-13,-3.73873020481597));
#2726=CARTESIAN_POINT('',(60.9647489474622,1.66533453693773E-13,81.1119190693219));
#2727=CARTESIAN_POINT('Origin',(133.453989983444,0.,57.6225611805379));
#2728=CARTESIAN_POINT('',(57.4875276588944,1.11022302462516E-13,84.9685467671164));
#2729=CARTESIAN_POINT('Origin',(39.2316144081271,1.66533453693773E-13,65.0127255748485));
#2730=CARTESIAN_POINT('',(33.0644120885454,1.66533453693773E-13,51.3530120545087));
#2731=CARTESIAN_POINT('',(49.6788956291876,1.11022302462516E-13,90.6418500222421));
#2732=CARTESIAN_POINT('',(25.2557800588381,0.,57.0263153096353));
#2733=CARTESIAN_POINT('Origin',(36.3411692885802,1.66533453693773E-13,67.1127568790624));
#2734=CARTESIAN_POINT('',(-49.2861156657315,-5.55111512312578E-14,90.6418500222435));
#2735=CARTESIAN_POINT('Origin',(-35.9483893251246,1.11022302462516E-13,
67.1127568790628));
#2736=CARTESIAN_POINT('',(-24.8630000953821,1.11022302462516E-13,57.0263153096384));
#2737=CARTESIAN_POINT('',(-57.0947476954385,1.11022302462516E-13,84.9685467671164));
#2738=CARTESIAN_POINT('',(-32.6716321250895,0.,51.3530120545105));
#2739=CARTESIAN_POINT('',(-60.5719689840063,1.11022302462516E-13,81.1119190693219));
#2740=CARTESIAN_POINT('Origin',(-38.8388344446712,1.11022302462516E-13,
65.0127255748476));
#2741=CARTESIAN_POINT('',(-88.2228802653845,-5.55111512312578E-14,-3.98883536926853));
#2742=CARTESIAN_POINT('Origin',(-133.061210019987,-5.55111512312578E-14,
57.6225611805379));
#2743=CARTESIAN_POINT('',(-87.6766180340772,-5.55111512312578E-14,-9.15277211013876));
#2744=CARTESIAN_POINT('Origin',(-61.17753657217,1.11022302462516E-13,-3.73873020481819));
#2745=CARTESIAN_POINT('',(-48.1591869300858,-5.55111512312578E-14,3.68721960007434));
#2746=CARTESIAN_POINT('',(-48.1591869300858,-5.55111512312578E-14,3.68721960007434));
#2747=CARTESIAN_POINT('',(-45.1765549003784,-5.55111512312578E-14,-5.4923778952074));
#2748=CARTESIAN_POINT('Origin',(-46.6678709152318,0.,-0.902579147564531));
#2749=CARTESIAN_POINT('',(-84.6939860043709,-5.55111512312578E-14,-18.332369605421));
#2750=CARTESIAN_POINT('',(-45.1765549003784,-5.55111512312578E-14,-5.4923778952074));
#2751=CARTESIAN_POINT('',(-82.1006355728287,-5.55111512312578E-14,-22.8311670701098));
#2752=CARTESIAN_POINT('Origin',(-60.07348477912,1.11022302462516E-13,-7.13665223247828));
#2753=CARTESIAN_POINT('',(-9.70961001827242,1.11022302462516E-13,-75.4263257814172));
#2754=CARTESIAN_POINT('Origin',(-82.1613360785705,-5.55111512312578E-14,
-99.0311428932596));
#2755=CARTESIAN_POINT('',(-4.62961001827211,1.66533453693773E-13,-76.5025437375311));
#2756=CARTESIAN_POINT('Origin',(-1.59000334476844,1.11022302462516E-13,
-49.6273886803462));
#2757=CARTESIAN_POINT('',(-4.62961001827178,0.,-34.9514577327459));
#2758=CARTESIAN_POINT('Origin',(0.196389981728107,12.7,-34.9514577327463));
#2759=CARTESIAN_POINT('',(-4.62961001827178,12.7,-34.9514577327459));
#2760=CARTESIAN_POINT('',(5.02238998172821,12.7,-34.9514577327463));
#2761=CARTESIAN_POINT('Origin',(-4.62961001827178,12.7,-34.9514577327459));
#2762=CARTESIAN_POINT('',(-4.62961001827222,12.7000000000002,-76.5025437375311));
#2763=CARTESIAN_POINT('Origin',(-1.59000334476855,12.7000000000001,-49.6273886803462));
#2764=CARTESIAN_POINT('',(-9.70961001827242,12.7000000000001,-75.4263257814172));
#2765=CARTESIAN_POINT('Origin',(-82.1613360785705,12.6999999999999,-99.0311428932596));
#2766=CARTESIAN_POINT('',(-82.1006355728287,12.6999999999999,-22.8311670701098));
#2767=CARTESIAN_POINT('Origin',(-60.07348477912,12.7000000000001,-7.13665223247828));
#2768=CARTESIAN_POINT('',(-84.6939860043709,12.6999999999999,-18.332369605421));
#2769=CARTESIAN_POINT('Origin',(-45.1765549003784,12.7,-5.4923778952074));
#2770=CARTESIAN_POINT('',(-45.1765549003784,12.7,-5.4923778952074));
#2771=CARTESIAN_POINT('Origin',(-46.6678709152318,12.7,-0.902579147566751));
#2772=CARTESIAN_POINT('',(-48.1591869300858,12.7,3.68721960007434));
#2773=CARTESIAN_POINT('Origin',(-48.1591869300858,12.7,3.68721960007434));
#2774=CARTESIAN_POINT('',(-87.6766180340772,12.6999999999999,-9.15277211013876));
#2775=CARTESIAN_POINT('Origin',(-61.17753657217,12.7000000000001,-3.73873020481819));
#2776=CARTESIAN_POINT('',(-88.2228802653845,12.6999999999999,-3.98883536926853));
#2777=CARTESIAN_POINT('Origin',(-133.061210019987,12.7,57.6225611805379));
#2778=CARTESIAN_POINT('',(-60.5719689840063,12.7000000000001,81.1119190693219));
#2779=CARTESIAN_POINT('Origin',(-38.8388344446712,12.7000000000001,65.0127255748467));
#2780=CARTESIAN_POINT('',(-57.0947476954385,12.7000000000001,84.9685467671164));
#2781=CARTESIAN_POINT('Origin',(-32.6716321250896,12.7,51.35301205451));
#2782=CARTESIAN_POINT('Origin',(-24.8630000953821,12.7000000000001,57.0263153096384));
#2783=CARTESIAN_POINT('',(-49.2861156657315,12.7,90.6418500222435));
#2784=CARTESIAN_POINT('Origin',(-35.9483893251246,12.7000000000001,67.1127568790628));
#2785=CARTESIAN_POINT('Origin',(36.3411692885806,12.7000000000002,67.1127568790633));
#2786=CARTESIAN_POINT('',(49.6788956291876,12.7000000000001,90.6418500222421));
#2787=CARTESIAN_POINT('Origin',(25.2557800588381,12.7,57.0263153096353));
#2788=CARTESIAN_POINT('Origin',(33.0644120885452,12.7000000000002,51.3530120545092));
#2789=CARTESIAN_POINT('',(57.4875276588944,12.7000000000001,84.9685467671164));
#2790=CARTESIAN_POINT('Origin',(39.2316144081271,12.7000000000002,65.0127255748485));
#2791=CARTESIAN_POINT('',(60.964748947462,12.7000000000002,81.1119190693224));
#2792=CARTESIAN_POINT('Origin',(133.453989983443,12.7,57.6225611805374));
#2793=CARTESIAN_POINT('',(88.61566022884,12.7,-3.98883536926897));
#2794=CARTESIAN_POINT('Origin',(61.5703165356259,12.7000000000001,-3.73873020481819));
#2795=CARTESIAN_POINT('',(88.0693979975334,12.7,-9.15277211014009));
#2796=CARTESIAN_POINT('Origin',(48.5519668935416,12.7000000000002,3.6872196000739));
#2797=CARTESIAN_POINT('',(48.5519668935416,12.7000000000002,3.6872196000739));
#2798=CARTESIAN_POINT('Origin',(47.0606508786874,12.7000000000001,-0.902579147566307));
#2799=CARTESIAN_POINT('',(45.5693348638345,12.7000000000002,-5.49237789520696));
#2800=CARTESIAN_POINT('Origin',(45.5693348638345,12.7000000000002,-5.49237789520696));
#2801=CARTESIAN_POINT('',(85.0867659678262,12.7000000000001,-18.3323696054205));
#2802=CARTESIAN_POINT('Origin',(60.4662647425757,12.7000000000001,-7.13665223247784));
#2803=CARTESIAN_POINT('',(82.4934155362843,12.7000000000002,-22.831167070108));
#2804=CARTESIAN_POINT('Origin',(82.5541160420259,12.7,-99.0311428932582));
#2805=CARTESIAN_POINT('',(10.1023899817279,12.7000000000002,-75.4263257814172));
#2806=CARTESIAN_POINT('Origin',(1.98278330822388,12.7000000000001,-49.6273886803467));
#2807=CARTESIAN_POINT('',(5.02238998172799,12.7000000000001,-76.5025437375311));
#2808=CARTESIAN_POINT('Origin',(5.02238998172821,12.7,-34.9514577327463));
#2809=CARTESIAN_POINT('Origin',(0.196389981728107,9.52499999999995,14.3245422672531));
#2830=UNCERTAINTY_MEASURE_WITH_UNIT(LENGTH_MEASURE(0.01),#2841,
'DISTANCE_ACCURACY_VALUE',
'Maximum model space distance between geometric entities at asserted c
onnectivities');
#2832=UNCERTAINTY_MEASURE_WITH_UNIT(LENGTH_MEASURE(0.01),#2841,
'DISTANCE_ACCURACY_VALUE',
'Maximum model space distance between geometric entities at asserted c
onnectivities');
#2838=(
GEOMETRIC_REPRESENTATION_CONTEXT(3)
GLOBAL_UNCERTAINTY_ASSIGNED_CONTEXT((#2830))
GLOBAL_UNIT_ASSIGNED_CONTEXT((#2841,#2843,#2844))
REPRESENTATION_CONTEXT('','3D')
);
#2840=(
GEOMETRIC_REPRESENTATION_CONTEXT(3)
GLOBAL_UNCERTAINTY_ASSIGNED_CONTEXT((#2832))
GLOBAL_UNIT_ASSIGNED_CONTEXT((#2841,#2843,#2844))
REPRESENTATION_CONTEXT('','3D')
);
#2841=(
LENGTH_UNIT()
NAMED_UNIT(*)
SI_UNIT(.MILLI.,.METRE.)
);
#2843=(
NAMED_UNIT(*)
PLANE_ANGLE_UNIT()
SI_UNIT($,.RADIAN.)
);
#2844=(
NAMED_UNIT(*)
SI_UNIT($,.STERADIAN.)
SOLID_ANGLE_UNIT()
);
#2850=SHAPE_DEFINITION_REPRESENTATION(#2857,#2870);
#2857=PRODUCT_DEFINITION_SHAPE('',$,#2878);
#2870=SHAPE_REPRESENTATION('',(#1749),#2838);
#2872=PRODUCT_DEFINITION_CONTEXT('part definition',#2895,'design');
#2878=PRODUCT_DEFINITION('Geneva Wheel','Geneva Wheel',#2885,#2872);
#2885=PRODUCT_DEFINITION_FORMATION('',$,#2902);
#2895=APPLICATION_CONTEXT(
'Core Data for Automotive Mechanical Design Process');
#2896=PRODUCT_CONTEXT('part definition',#2895,'mechanical');
#2902=PRODUCT('Geneva Wheel','Geneva Wheel',$,(#2896));
#2905=PRESENTATION_STYLE_ASSIGNMENT((#2907));
#2907=SURFACE_STYLE_USAGE(.BOTH.,#2909);
#2909=SURFACE_SIDE_STYLE('',(#2911));
#2911=SURFACE_STYLE_FILL_AREA(#2913);
#2913=FILL_AREA_STYLE('Opaque(202,209,238)',(#2915));
#2915=FILL_AREA_STYLE_COLOUR('Opaque(202,209,238)',#2917);
#2917=COLOUR_RGB('Opaque(202,209,238)', 0.66274510, 0.83137255, 0.94901961);
ENDSEC;
END-ISO-10303-21;
